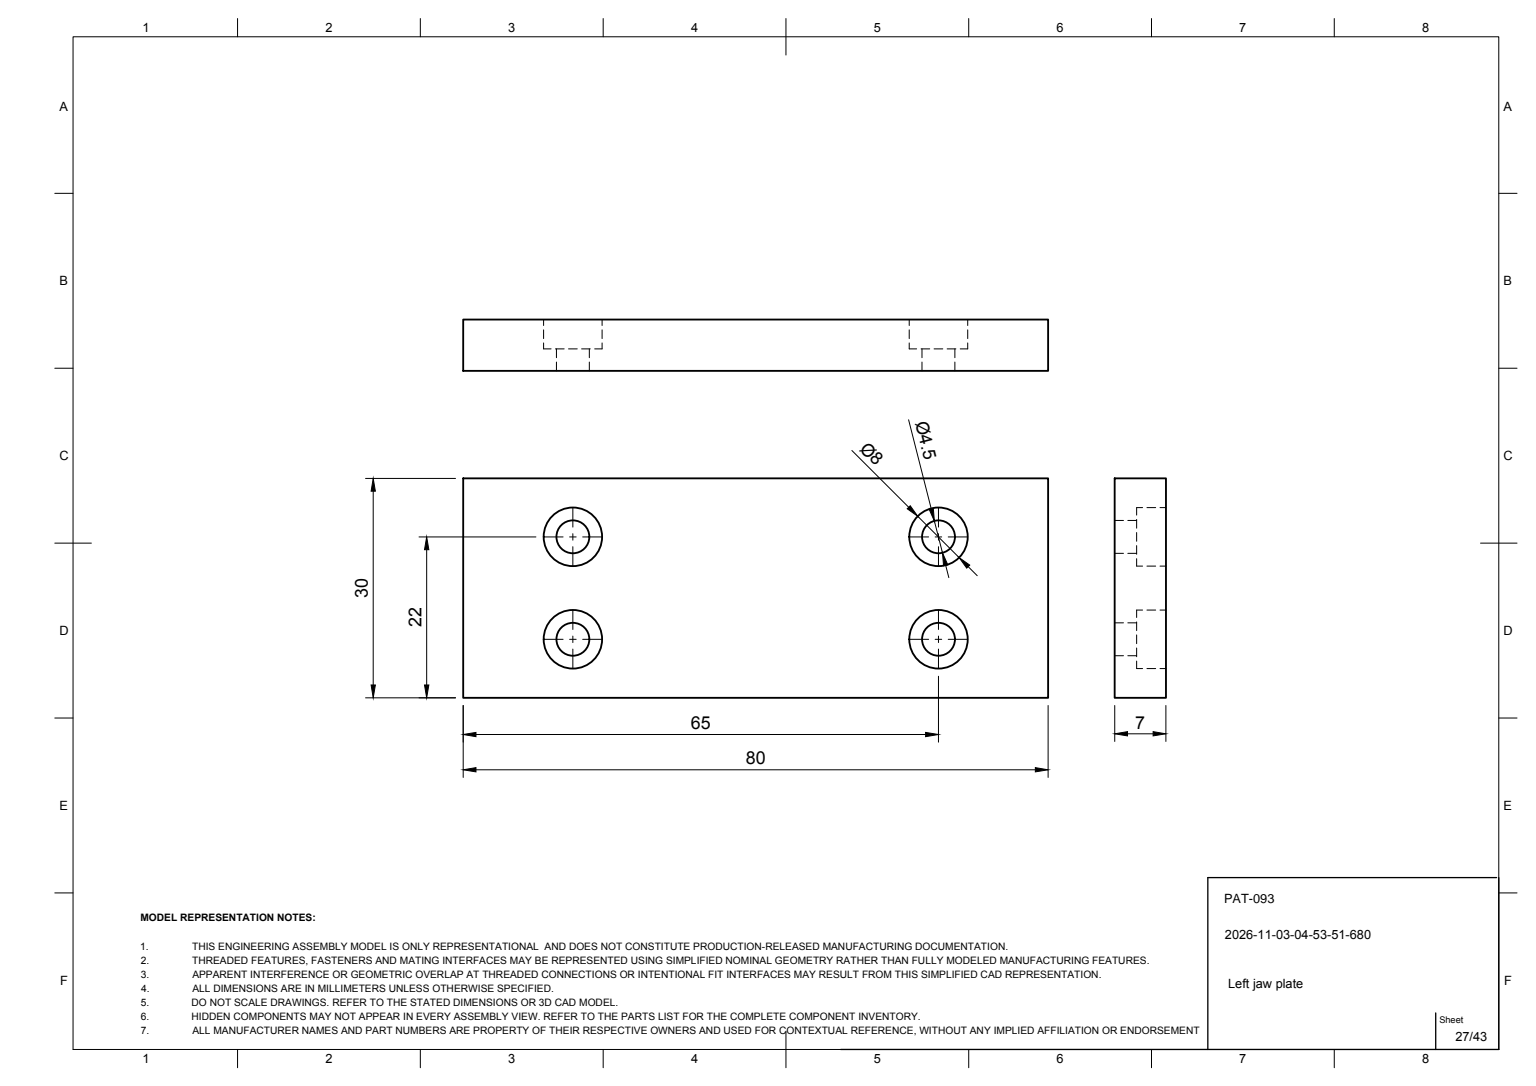
ISO-10303-21;
HEADER;
/* Generated by software containing ST-Developer
 * from STEP Tools, Inc. (www.steptools.com) 
 */

FILE_DESCRIPTION(
/* description */ ('Self-centering screw clamp'),
/* implementation_level */ '2;1');

FILE_NAME(
/* name */ 'Left jaw plate.step',
/* time_stamp */ '2026-10-28T03:25:31-07:00',
/* author */ (''),
/* organization */ (''),
/* preprocessor_version */ 'ST-DEVELOPER v20.2',
/* originating_system */ 'Autodesk Translation Framework v15.17.0.0',
/* authorisation */ '');

FILE_SCHEMA (('AUTOMOTIVE_DESIGN { 1 0 10303 214 3 1 1 }'));
ENDSEC;

DATA;
#10=MECHANICAL_DESIGN_GEOMETRIC_PRESENTATION_REPRESENTATION('',(#654),#16799);
#565=SHAPE_REPRESENTATION_RELATIONSHIP('SRR','None',#17040,#606);
#606=ADVANCED_BREP_SHAPE_REPRESENTATION('',(#702),#16778);
#654=STYLED_ITEM('',(#17340),#702);
#702=MANIFOLD_SOLID_BREP('Body1',#9105);
#904=FACE_BOUND('',#2255,.T.);
#905=FACE_BOUND('',#2258,.T.);
#906=FACE_BOUND('',#2261,.T.);
#907=FACE_BOUND('',#2264,.T.);
#908=FACE_BOUND('',#2271,.T.);
#909=FACE_BOUND('',#2272,.T.);
#910=FACE_BOUND('',#2273,.T.);
#911=FACE_BOUND('',#2274,.T.);
#912=FACE_BOUND('',#2277,.T.);
#913=FACE_BOUND('',#2278,.T.);
#914=FACE_BOUND('',#2279,.T.);
#915=FACE_BOUND('',#2280,.T.);
#1151=PLANE('',#10224);
#1152=PLANE('',#10229);
#1153=PLANE('',#10234);
#1154=PLANE('',#10239);
#1155=PLANE('',#10249);
#1156=PLANE('',#10250);
#1157=PLANE('',#10251);
#1158=PLANE('',#10252);
#1159=PLANE('',#10253);
#1160=PLANE('',#10254);
#1563=FACE_OUTER_BOUND('',#2253,.T.);
#1564=FACE_OUTER_BOUND('',#2254,.T.);
#1565=FACE_OUTER_BOUND('',#2256,.T.);
#1566=FACE_OUTER_BOUND('',#2257,.T.);
#1567=FACE_OUTER_BOUND('',#2259,.T.);
#1568=FACE_OUTER_BOUND('',#2260,.T.);
#1569=FACE_OUTER_BOUND('',#2262,.T.);
#1570=FACE_OUTER_BOUND('',#2263,.T.);
#1571=FACE_OUTER_BOUND('',#2265,.T.);
#1572=FACE_OUTER_BOUND('',#2266,.T.);
#1573=FACE_OUTER_BOUND('',#2267,.T.);
#1574=FACE_OUTER_BOUND('',#2268,.T.);
#1575=FACE_OUTER_BOUND('',#2269,.T.);
#1576=FACE_OUTER_BOUND('',#2270,.T.);
#1577=FACE_OUTER_BOUND('',#2275,.T.);
#1578=FACE_OUTER_BOUND('',#2276,.T.);
#1579=FACE_OUTER_BOUND('',#2281,.T.);
#1580=FACE_OUTER_BOUND('',#2282,.T.);
#2253=EDGE_LOOP('',(#7479,#7480,#7481,#7482));
#2254=EDGE_LOOP('',(#7483));
#2255=EDGE_LOOP('',(#7484));
#2256=EDGE_LOOP('',(#7485,#7486,#7487,#7488));
#2257=EDGE_LOOP('',(#7489));
#2258=EDGE_LOOP('',(#7490));
#2259=EDGE_LOOP('',(#7491,#7492,#7493,#7494));
#2260=EDGE_LOOP('',(#7495));
#2261=EDGE_LOOP('',(#7496));
#2262=EDGE_LOOP('',(#7497,#7498,#7499,#7500));
#2263=EDGE_LOOP('',(#7501));
#2264=EDGE_LOOP('',(#7502));
#2265=EDGE_LOOP('',(#7503,#7504,#7505,#7506));
#2266=EDGE_LOOP('',(#7507,#7508,#7509,#7510));
#2267=EDGE_LOOP('',(#7511,#7512,#7513,#7514));
#2268=EDGE_LOOP('',(#7515,#7516,#7517,#7518));
#2269=EDGE_LOOP('',(#7519,#7520,#7521,#7522));
#2270=EDGE_LOOP('',(#7523,#7524,#7525,#7526));
#2271=EDGE_LOOP('',(#7527));
#2272=EDGE_LOOP('',(#7528));
#2273=EDGE_LOOP('',(#7529));
#2274=EDGE_LOOP('',(#7530));
#2275=EDGE_LOOP('',(#7531,#7532,#7533,#7534));
#2276=EDGE_LOOP('',(#7535,#7536,#7537,#7538));
#2277=EDGE_LOOP('',(#7539));
#2278=EDGE_LOOP('',(#7540));
#2279=EDGE_LOOP('',(#7541));
#2280=EDGE_LOOP('',(#7542));
#2281=EDGE_LOOP('',(#7543,#7544,#7545,#7546));
#2282=EDGE_LOOP('',(#7547,#7548,#7549,#7550));
#2914=LINE('',#15518,#3487);
#2915=LINE('',#15527,#3488);
#2916=LINE('',#15536,#3489);
#2917=LINE('',#15545,#3490);
#2918=LINE('',#15553,#3491);
#2919=LINE('',#15557,#3492);
#2920=LINE('',#15561,#3493);
#2921=LINE('',#15565,#3494);
#2922=LINE('',#15569,#3495);
#2923=LINE('',#15571,#3496);
#2924=LINE('',#15573,#3497);
#2925=LINE('',#15574,#3498);
#2926=LINE('',#15577,#3499);
#2927=LINE('',#15579,#3500);
#2928=LINE('',#15580,#3501);
#2929=LINE('',#15583,#3502);
#2930=LINE('',#15585,#3503);
#2931=LINE('',#15586,#3504);
#2932=LINE('',#15588,#3505);
#2933=LINE('',#15589,#3506);
#3487=VECTOR('',#12381,0.4);
#3488=VECTOR('',#12392,0.4);
#3489=VECTOR('',#12403,0.4);
#3490=VECTOR('',#12414,0.4);
#3491=VECTOR('',#12425,0.225);
#3492=VECTOR('',#12430,0.225);
#3493=VECTOR('',#12435,0.225);
#3494=VECTOR('',#12440,0.225);
#3495=VECTOR('',#12443,1.);
#3496=VECTOR('',#12444,1.);
#3497=VECTOR('',#12445,1.);
#3498=VECTOR('',#12446,1.);
#3499=VECTOR('',#12449,1.);
#3500=VECTOR('',#12450,1.);
#3501=VECTOR('',#12451,1.);
#3502=VECTOR('',#12454,1.);
#3503=VECTOR('',#12455,1.);
#3504=VECTOR('',#12456,1.);
#3505=VECTOR('',#12459,1.);
#3506=VECTOR('',#12460,1.);
#4044=CIRCLE('',#10222,0.4);
#4045=CIRCLE('',#10223,0.4);
#4046=CIRCLE('',#10225,0.225);
#4047=CIRCLE('',#10227,0.4);
#4048=CIRCLE('',#10228,0.4);
#4049=CIRCLE('',#10230,0.225);
#4050=CIRCLE('',#10232,0.4);
#4051=CIRCLE('',#10233,0.4);
#4052=CIRCLE('',#10235,0.225);
#4053=CIRCLE('',#10237,0.4);
#4054=CIRCLE('',#10238,0.4);
#4055=CIRCLE('',#10240,0.225);
#4056=CIRCLE('',#10242,0.225);
#4057=CIRCLE('',#10244,0.225);
#4058=CIRCLE('',#10246,0.225);
#4059=CIRCLE('',#10248,0.225);
#4687=VERTEX_POINT('',#15515);
#4688=VERTEX_POINT('',#15517);
#4689=VERTEX_POINT('',#15521);
#4690=VERTEX_POINT('',#15524);
#4691=VERTEX_POINT('',#15526);
#4692=VERTEX_POINT('',#15530);
#4693=VERTEX_POINT('',#15533);
#4694=VERTEX_POINT('',#15535);
#4695=VERTEX_POINT('',#15539);
#4696=VERTEX_POINT('',#15542);
#4697=VERTEX_POINT('',#15544);
#4698=VERTEX_POINT('',#15548);
#4699=VERTEX_POINT('',#15551);
#4700=VERTEX_POINT('',#15555);
#4701=VERTEX_POINT('',#15559);
#4702=VERTEX_POINT('',#15563);
#4703=VERTEX_POINT('',#15567);
#4704=VERTEX_POINT('',#15568);
#4705=VERTEX_POINT('',#15570);
#4706=VERTEX_POINT('',#15572);
#4707=VERTEX_POINT('',#15576);
#4708=VERTEX_POINT('',#15578);
#4709=VERTEX_POINT('',#15582);
#4710=VERTEX_POINT('',#15584);
#5664=EDGE_CURVE('',#4687,#4687,#4044,.T.);
#5665=EDGE_CURVE('',#4687,#4688,#2914,.T.);
#5666=EDGE_CURVE('',#4688,#4688,#4045,.T.);
#5667=EDGE_CURVE('',#4689,#4689,#4046,.T.);
#5668=EDGE_CURVE('',#4690,#4690,#4047,.T.);
#5669=EDGE_CURVE('',#4690,#4691,#2915,.T.);
#5670=EDGE_CURVE('',#4691,#4691,#4048,.T.);
#5671=EDGE_CURVE('',#4692,#4692,#4049,.T.);
#5672=EDGE_CURVE('',#4693,#4693,#4050,.T.);
#5673=EDGE_CURVE('',#4693,#4694,#2916,.T.);
#5674=EDGE_CURVE('',#4694,#4694,#4051,.T.);
#5675=EDGE_CURVE('',#4695,#4695,#4052,.T.);
#5676=EDGE_CURVE('',#4696,#4696,#4053,.T.);
#5677=EDGE_CURVE('',#4696,#4697,#2917,.T.);
#5678=EDGE_CURVE('',#4697,#4697,#4054,.T.);
#5679=EDGE_CURVE('',#4698,#4698,#4055,.T.);
#5680=EDGE_CURVE('',#4699,#4699,#4056,.T.);
#5681=EDGE_CURVE('',#4699,#4689,#2918,.T.);
#5682=EDGE_CURVE('',#4700,#4700,#4057,.T.);
#5683=EDGE_CURVE('',#4700,#4692,#2919,.T.);
#5684=EDGE_CURVE('',#4701,#4701,#4058,.T.);
#5685=EDGE_CURVE('',#4701,#4695,#2920,.T.);
#5686=EDGE_CURVE('',#4702,#4702,#4059,.T.);
#5687=EDGE_CURVE('',#4702,#4698,#2921,.T.);
#5688=EDGE_CURVE('',#4703,#4704,#2922,.T.);
#5689=EDGE_CURVE('',#4704,#4705,#2923,.T.);
#5690=EDGE_CURVE('',#4706,#4705,#2924,.T.);
#5691=EDGE_CURVE('',#4703,#4706,#2925,.T.);
#5692=EDGE_CURVE('',#4707,#4703,#2926,.T.);
#5693=EDGE_CURVE('',#4708,#4706,#2927,.T.);
#5694=EDGE_CURVE('',#4707,#4708,#2928,.T.);
#5695=EDGE_CURVE('',#4709,#4707,#2929,.T.);
#5696=EDGE_CURVE('',#4710,#4708,#2930,.T.);
#5697=EDGE_CURVE('',#4709,#4710,#2931,.T.);
#5698=EDGE_CURVE('',#4704,#4709,#2932,.T.);
#5699=EDGE_CURVE('',#4705,#4710,#2933,.T.);
#7479=ORIENTED_EDGE('',*,*,#5664,.F.);
#7480=ORIENTED_EDGE('',*,*,#5665,.T.);
#7481=ORIENTED_EDGE('',*,*,#5666,.F.);
#7482=ORIENTED_EDGE('',*,*,#5665,.F.);
#7483=ORIENTED_EDGE('',*,*,#5664,.T.);
#7484=ORIENTED_EDGE('',*,*,#5667,.F.);
#7485=ORIENTED_EDGE('',*,*,#5668,.F.);
#7486=ORIENTED_EDGE('',*,*,#5669,.T.);
#7487=ORIENTED_EDGE('',*,*,#5670,.F.);
#7488=ORIENTED_EDGE('',*,*,#5669,.F.);
#7489=ORIENTED_EDGE('',*,*,#5668,.T.);
#7490=ORIENTED_EDGE('',*,*,#5671,.F.);
#7491=ORIENTED_EDGE('',*,*,#5672,.F.);
#7492=ORIENTED_EDGE('',*,*,#5673,.T.);
#7493=ORIENTED_EDGE('',*,*,#5674,.F.);
#7494=ORIENTED_EDGE('',*,*,#5673,.F.);
#7495=ORIENTED_EDGE('',*,*,#5672,.T.);
#7496=ORIENTED_EDGE('',*,*,#5675,.F.);
#7497=ORIENTED_EDGE('',*,*,#5676,.F.);
#7498=ORIENTED_EDGE('',*,*,#5677,.T.);
#7499=ORIENTED_EDGE('',*,*,#5678,.F.);
#7500=ORIENTED_EDGE('',*,*,#5677,.F.);
#7501=ORIENTED_EDGE('',*,*,#5676,.T.);
#7502=ORIENTED_EDGE('',*,*,#5679,.F.);
#7503=ORIENTED_EDGE('',*,*,#5680,.F.);
#7504=ORIENTED_EDGE('',*,*,#5681,.T.);
#7505=ORIENTED_EDGE('',*,*,#5667,.T.);
#7506=ORIENTED_EDGE('',*,*,#5681,.F.);
#7507=ORIENTED_EDGE('',*,*,#5682,.F.);
#7508=ORIENTED_EDGE('',*,*,#5683,.T.);
#7509=ORIENTED_EDGE('',*,*,#5671,.T.);
#7510=ORIENTED_EDGE('',*,*,#5683,.F.);
#7511=ORIENTED_EDGE('',*,*,#5684,.F.);
#7512=ORIENTED_EDGE('',*,*,#5685,.T.);
#7513=ORIENTED_EDGE('',*,*,#5675,.T.);
#7514=ORIENTED_EDGE('',*,*,#5685,.F.);
#7515=ORIENTED_EDGE('',*,*,#5686,.F.);
#7516=ORIENTED_EDGE('',*,*,#5687,.T.);
#7517=ORIENTED_EDGE('',*,*,#5679,.T.);
#7518=ORIENTED_EDGE('',*,*,#5687,.F.);
#7519=ORIENTED_EDGE('',*,*,#5688,.T.);
#7520=ORIENTED_EDGE('',*,*,#5689,.T.);
#7521=ORIENTED_EDGE('',*,*,#5690,.F.);
#7522=ORIENTED_EDGE('',*,*,#5691,.F.);
#7523=ORIENTED_EDGE('',*,*,#5692,.T.);
#7524=ORIENTED_EDGE('',*,*,#5691,.T.);
#7525=ORIENTED_EDGE('',*,*,#5693,.F.);
#7526=ORIENTED_EDGE('',*,*,#5694,.F.);
#7527=ORIENTED_EDGE('',*,*,#5678,.T.);
#7528=ORIENTED_EDGE('',*,*,#5674,.T.);
#7529=ORIENTED_EDGE('',*,*,#5670,.T.);
#7530=ORIENTED_EDGE('',*,*,#5666,.T.);
#7531=ORIENTED_EDGE('',*,*,#5695,.T.);
#7532=ORIENTED_EDGE('',*,*,#5694,.T.);
#7533=ORIENTED_EDGE('',*,*,#5696,.F.);
#7534=ORIENTED_EDGE('',*,*,#5697,.F.);
#7535=ORIENTED_EDGE('',*,*,#5698,.T.);
#7536=ORIENTED_EDGE('',*,*,#5697,.T.);
#7537=ORIENTED_EDGE('',*,*,#5699,.F.);
#7538=ORIENTED_EDGE('',*,*,#5689,.F.);
#7539=ORIENTED_EDGE('',*,*,#5680,.T.);
#7540=ORIENTED_EDGE('',*,*,#5682,.T.);
#7541=ORIENTED_EDGE('',*,*,#5684,.T.);
#7542=ORIENTED_EDGE('',*,*,#5686,.T.);
#7543=ORIENTED_EDGE('',*,*,#5699,.T.);
#7544=ORIENTED_EDGE('',*,*,#5696,.T.);
#7545=ORIENTED_EDGE('',*,*,#5693,.T.);
#7546=ORIENTED_EDGE('',*,*,#5690,.T.);
#7547=ORIENTED_EDGE('',*,*,#5698,.F.);
#7548=ORIENTED_EDGE('',*,*,#5688,.F.);
#7549=ORIENTED_EDGE('',*,*,#5692,.F.);
#7550=ORIENTED_EDGE('',*,*,#5695,.F.);
#8488=CYLINDRICAL_SURFACE('',#10221,0.4);
#8489=CYLINDRICAL_SURFACE('',#10226,0.4);
#8490=CYLINDRICAL_SURFACE('',#10231,0.4);
#8491=CYLINDRICAL_SURFACE('',#10236,0.4);
#8492=CYLINDRICAL_SURFACE('',#10241,0.225);
#8493=CYLINDRICAL_SURFACE('',#10243,0.225);
#8494=CYLINDRICAL_SURFACE('',#10245,0.225);
#8495=CYLINDRICAL_SURFACE('',#10247,0.225);
#8861=ADVANCED_FACE('',(#1563),#8488,.F.);
#8862=ADVANCED_FACE('',(#1564,#904),#1151,.T.);
#8863=ADVANCED_FACE('',(#1565),#8489,.F.);
#8864=ADVANCED_FACE('',(#1566,#905),#1152,.T.);
#8865=ADVANCED_FACE('',(#1567),#8490,.F.);
#8866=ADVANCED_FACE('',(#1568,#906),#1153,.T.);
#8867=ADVANCED_FACE('',(#1569),#8491,.F.);
#8868=ADVANCED_FACE('',(#1570,#907),#1154,.T.);
#8869=ADVANCED_FACE('',(#1571),#8492,.F.);
#8870=ADVANCED_FACE('',(#1572),#8493,.F.);
#8871=ADVANCED_FACE('',(#1573),#8494,.F.);
#8872=ADVANCED_FACE('',(#1574),#8495,.F.);
#8873=ADVANCED_FACE('',(#1575),#1155,.T.);
#8874=ADVANCED_FACE('',(#1576,#908,#909,#910,#911),#1156,.T.);
#8875=ADVANCED_FACE('',(#1577),#1157,.T.);
#8876=ADVANCED_FACE('',(#1578,#912,#913,#914,#915),#1158,.T.);
#8877=ADVANCED_FACE('',(#1579),#1159,.T.);
#8878=ADVANCED_FACE('',(#1580),#1160,.F.);
#9105=CLOSED_SHELL('',(#8861,#8862,#8863,#8864,#8865,#8866,#8867,#8868,
#8869,#8870,#8871,#8872,#8873,#8874,#8875,#8876,#8877,#8878));
#10220=AXIS2_PLACEMENT_3D('',#15513,#12375,#12376);
#10221=AXIS2_PLACEMENT_3D('',#15514,#12377,#12378);
#10222=AXIS2_PLACEMENT_3D('',#15516,#12379,#12380);
#10223=AXIS2_PLACEMENT_3D('',#15519,#12382,#12383);
#10224=AXIS2_PLACEMENT_3D('',#15520,#12384,#12385);
#10225=AXIS2_PLACEMENT_3D('',#15522,#12386,#12387);
#10226=AXIS2_PLACEMENT_3D('',#15523,#12388,#12389);
#10227=AXIS2_PLACEMENT_3D('',#15525,#12390,#12391);
#10228=AXIS2_PLACEMENT_3D('',#15528,#12393,#12394);
#10229=AXIS2_PLACEMENT_3D('',#15529,#12395,#12396);
#10230=AXIS2_PLACEMENT_3D('',#15531,#12397,#12398);
#10231=AXIS2_PLACEMENT_3D('',#15532,#12399,#12400);
#10232=AXIS2_PLACEMENT_3D('',#15534,#12401,#12402);
#10233=AXIS2_PLACEMENT_3D('',#15537,#12404,#12405);
#10234=AXIS2_PLACEMENT_3D('',#15538,#12406,#12407);
#10235=AXIS2_PLACEMENT_3D('',#15540,#12408,#12409);
#10236=AXIS2_PLACEMENT_3D('',#15541,#12410,#12411);
#10237=AXIS2_PLACEMENT_3D('',#15543,#12412,#12413);
#10238=AXIS2_PLACEMENT_3D('',#15546,#12415,#12416);
#10239=AXIS2_PLACEMENT_3D('',#15547,#12417,#12418);
#10240=AXIS2_PLACEMENT_3D('',#15549,#12419,#12420);
#10241=AXIS2_PLACEMENT_3D('',#15550,#12421,#12422);
#10242=AXIS2_PLACEMENT_3D('',#15552,#12423,#12424);
#10243=AXIS2_PLACEMENT_3D('',#15554,#12426,#12427);
#10244=AXIS2_PLACEMENT_3D('',#15556,#12428,#12429);
#10245=AXIS2_PLACEMENT_3D('',#15558,#12431,#12432);
#10246=AXIS2_PLACEMENT_3D('',#15560,#12433,#12434);
#10247=AXIS2_PLACEMENT_3D('',#15562,#12436,#12437);
#10248=AXIS2_PLACEMENT_3D('',#15564,#12438,#12439);
#10249=AXIS2_PLACEMENT_3D('',#15566,#12441,#12442);
#10250=AXIS2_PLACEMENT_3D('',#15575,#12447,#12448);
#10251=AXIS2_PLACEMENT_3D('',#15581,#12452,#12453);
#10252=AXIS2_PLACEMENT_3D('',#15587,#12457,#12458);
#10253=AXIS2_PLACEMENT_3D('',#15590,#12461,#12462);
#10254=AXIS2_PLACEMENT_3D('',#15591,#12463,#12464);
#12375=DIRECTION('axis',(0.,0.,1.));
#12376=DIRECTION('refdir',(1.,0.,0.));
#12377=DIRECTION('center_axis',(1.,0.,0.));
#12378=DIRECTION('ref_axis',(0.,0.,-1.));
#12379=DIRECTION('center_axis',(1.,0.,0.));
#12380=DIRECTION('ref_axis',(0.,0.,-1.));
#12381=DIRECTION('',(1.,0.,0.));
#12382=DIRECTION('center_axis',(-1.,0.,0.));
#12383=DIRECTION('ref_axis',(0.,0.,-1.));
#12384=DIRECTION('center_axis',(1.,0.,0.));
#12385=DIRECTION('ref_axis',(0.,0.,-1.));
#12386=DIRECTION('center_axis',(1.,0.,0.));
#12387=DIRECTION('ref_axis',(0.,0.,-1.));
#12388=DIRECTION('center_axis',(1.,0.,0.));
#12389=DIRECTION('ref_axis',(0.,0.,-1.));
#12390=DIRECTION('center_axis',(1.,0.,0.));
#12391=DIRECTION('ref_axis',(0.,0.,-1.));
#12392=DIRECTION('',(1.,0.,0.));
#12393=DIRECTION('center_axis',(-1.,0.,0.));
#12394=DIRECTION('ref_axis',(0.,0.,-1.));
#12395=DIRECTION('center_axis',(1.,0.,0.));
#12396=DIRECTION('ref_axis',(0.,0.,-1.));
#12397=DIRECTION('center_axis',(1.,0.,0.));
#12398=DIRECTION('ref_axis',(0.,0.,-1.));
#12399=DIRECTION('center_axis',(1.,0.,0.));
#12400=DIRECTION('ref_axis',(0.,0.,-1.));
#12401=DIRECTION('center_axis',(1.,0.,0.));
#12402=DIRECTION('ref_axis',(0.,0.,-1.));
#12403=DIRECTION('',(1.,0.,0.));
#12404=DIRECTION('center_axis',(-1.,0.,0.));
#12405=DIRECTION('ref_axis',(0.,0.,-1.));
#12406=DIRECTION('center_axis',(1.,0.,0.));
#12407=DIRECTION('ref_axis',(0.,0.,-1.));
#12408=DIRECTION('center_axis',(1.,0.,0.));
#12409=DIRECTION('ref_axis',(0.,0.,-1.));
#12410=DIRECTION('center_axis',(1.,0.,0.));
#12411=DIRECTION('ref_axis',(0.,0.,-1.));
#12412=DIRECTION('center_axis',(1.,0.,0.));
#12413=DIRECTION('ref_axis',(0.,0.,-1.));
#12414=DIRECTION('',(1.,0.,0.));
#12415=DIRECTION('center_axis',(-1.,0.,0.));
#12416=DIRECTION('ref_axis',(0.,0.,-1.));
#12417=DIRECTION('center_axis',(1.,0.,0.));
#12418=DIRECTION('ref_axis',(0.,0.,-1.));
#12419=DIRECTION('center_axis',(1.,0.,0.));
#12420=DIRECTION('ref_axis',(0.,0.,-1.));
#12421=DIRECTION('center_axis',(1.,0.,0.));
#12422=DIRECTION('ref_axis',(0.,0.,-1.));
#12423=DIRECTION('center_axis',(1.,0.,0.));
#12424=DIRECTION('ref_axis',(0.,0.,-1.));
#12425=DIRECTION('',(1.,0.,0.));
#12426=DIRECTION('center_axis',(1.,0.,0.));
#12427=DIRECTION('ref_axis',(0.,0.,-1.));
#12428=DIRECTION('center_axis',(1.,0.,0.));
#12429=DIRECTION('ref_axis',(0.,0.,-1.));
#12430=DIRECTION('',(1.,0.,0.));
#12431=DIRECTION('center_axis',(1.,0.,0.));
#12432=DIRECTION('ref_axis',(0.,0.,-1.));
#12433=DIRECTION('center_axis',(1.,0.,0.));
#12434=DIRECTION('ref_axis',(0.,0.,-1.));
#12435=DIRECTION('',(1.,0.,0.));
#12436=DIRECTION('center_axis',(1.,0.,0.));
#12437=DIRECTION('ref_axis',(0.,0.,-1.));
#12438=DIRECTION('center_axis',(1.,0.,0.));
#12439=DIRECTION('ref_axis',(0.,0.,-1.));
#12440=DIRECTION('',(1.,0.,0.));
#12441=DIRECTION('center_axis',(0.,1.,0.));
#12442=DIRECTION('ref_axis',(-1.,0.,0.));
#12443=DIRECTION('',(-1.,0.,0.));
#12444=DIRECTION('',(0.,0.,1.));
#12445=DIRECTION('',(-1.,0.,0.));
#12446=DIRECTION('',(0.,0.,1.));
#12447=DIRECTION('center_axis',(1.,0.,0.));
#12448=DIRECTION('ref_axis',(0.,1.,0.));
#12449=DIRECTION('',(0.,1.,0.));
#12450=DIRECTION('',(0.,1.,0.));
#12451=DIRECTION('',(0.,0.,1.));
#12452=DIRECTION('center_axis',(0.,-1.,0.));
#12453=DIRECTION('ref_axis',(1.,0.,0.));
#12454=DIRECTION('',(1.,0.,0.));
#12455=DIRECTION('',(1.,0.,0.));
#12456=DIRECTION('',(0.,0.,1.));
#12457=DIRECTION('center_axis',(-1.,0.,0.));
#12458=DIRECTION('ref_axis',(0.,-1.,0.));
#12459=DIRECTION('',(0.,-1.,0.));
#12460=DIRECTION('',(0.,-1.,0.));
#12461=DIRECTION('center_axis',(0.,0.,1.));
#12462=DIRECTION('ref_axis',(1.,0.,0.));
#12463=DIRECTION('center_axis',(0.,0.,1.));
#12464=DIRECTION('ref_axis',(1.,0.,0.));
#15513=CARTESIAN_POINT('',(0.,0.,0.));
#15514=CARTESIAN_POINT('Origin',(-5.2,2.5,7.8));
#15515=CARTESIAN_POINT('',(-5.2,2.5,8.2));
#15516=CARTESIAN_POINT('Origin',(-5.2,2.5,7.8));
#15517=CARTESIAN_POINT('',(-4.8,2.5,8.2));
#15518=CARTESIAN_POINT('',(-5.2,2.5,8.2));
#15519=CARTESIAN_POINT('Origin',(-4.8,2.5,7.8));
#15520=CARTESIAN_POINT('Origin',(-5.2,2.5,7.8));
#15521=CARTESIAN_POINT('',(-5.2,2.5,8.025));
#15522=CARTESIAN_POINT('Origin',(-5.2,2.5,7.8));
#15523=CARTESIAN_POINT('Origin',(-5.2,-2.5,9.2));
#15524=CARTESIAN_POINT('',(-5.2,-2.5,9.6));
#15525=CARTESIAN_POINT('Origin',(-5.2,-2.5,9.2));
#15526=CARTESIAN_POINT('',(-4.8,-2.5,9.6));
#15527=CARTESIAN_POINT('',(-5.2,-2.5,9.6));
#15528=CARTESIAN_POINT('Origin',(-4.8,-2.5,9.2));
#15529=CARTESIAN_POINT('Origin',(-5.2,-2.5,9.2));
#15530=CARTESIAN_POINT('',(-5.2,-2.5,9.425));
#15531=CARTESIAN_POINT('Origin',(-5.2,-2.5,9.2));
#15532=CARTESIAN_POINT('Origin',(-5.2,-2.5,7.8));
#15533=CARTESIAN_POINT('',(-5.2,-2.5,8.2));
#15534=CARTESIAN_POINT('Origin',(-5.2,-2.5,7.8));
#15535=CARTESIAN_POINT('',(-4.8,-2.5,8.2));
#15536=CARTESIAN_POINT('',(-5.2,-2.5,8.2));
#15537=CARTESIAN_POINT('Origin',(-4.8,-2.5,7.8));
#15538=CARTESIAN_POINT('Origin',(-5.2,-2.5,7.8));
#15539=CARTESIAN_POINT('',(-5.2,-2.5,8.025));
#15540=CARTESIAN_POINT('Origin',(-5.2,-2.5,7.8));
#15541=CARTESIAN_POINT('Origin',(-5.2,2.5,9.2));
#15542=CARTESIAN_POINT('',(-5.2,2.5,9.6));
#15543=CARTESIAN_POINT('Origin',(-5.2,2.5,9.2));
#15544=CARTESIAN_POINT('',(-4.8,2.5,9.6));
#15545=CARTESIAN_POINT('',(-5.2,2.5,9.6));
#15546=CARTESIAN_POINT('Origin',(-4.8,2.5,9.2));
#15547=CARTESIAN_POINT('Origin',(-5.2,2.5,9.2));
#15548=CARTESIAN_POINT('',(-5.2,2.5,9.425));
#15549=CARTESIAN_POINT('Origin',(-5.2,2.5,9.2));
#15550=CARTESIAN_POINT('Origin',(-5.6,2.5,7.8));
#15551=CARTESIAN_POINT('',(-5.5,2.5,8.025));
#15552=CARTESIAN_POINT('Origin',(-5.5,2.5,7.8));
#15553=CARTESIAN_POINT('',(-5.6,2.5,8.025));
#15554=CARTESIAN_POINT('Origin',(-5.6,-2.5,9.2));
#15555=CARTESIAN_POINT('',(-5.5,-2.5,9.425));
#15556=CARTESIAN_POINT('Origin',(-5.5,-2.5,9.2));
#15557=CARTESIAN_POINT('',(-5.6,-2.5,9.425));
#15558=CARTESIAN_POINT('Origin',(-5.6,-2.5,7.8));
#15559=CARTESIAN_POINT('',(-5.5,-2.5,8.025));
#15560=CARTESIAN_POINT('Origin',(-5.5,-2.5,7.8));
#15561=CARTESIAN_POINT('',(-5.6,-2.5,8.025));
#15562=CARTESIAN_POINT('Origin',(-5.6,2.5,9.2));
#15563=CARTESIAN_POINT('',(-5.5,2.5,9.425));
#15564=CARTESIAN_POINT('Origin',(-5.5,2.5,9.2));
#15565=CARTESIAN_POINT('',(-5.6,2.5,9.425));
#15566=CARTESIAN_POINT('Origin',(-4.8,4.,7.));
#15567=CARTESIAN_POINT('',(-4.8,4.,7.));
#15568=CARTESIAN_POINT('',(-5.5,4.,7.));
#15569=CARTESIAN_POINT('',(-4.8,4.,7.));
#15570=CARTESIAN_POINT('',(-5.5,4.,10.));
#15571=CARTESIAN_POINT('',(-5.5,4.,7.));
#15572=CARTESIAN_POINT('',(-4.8,4.,10.));
#15573=CARTESIAN_POINT('',(-4.8,4.,10.));
#15574=CARTESIAN_POINT('',(-4.8,4.,7.));
#15575=CARTESIAN_POINT('Origin',(-4.8,-4.,7.));
#15576=CARTESIAN_POINT('',(-4.8,-4.,7.));
#15577=CARTESIAN_POINT('',(-4.8,-4.,7.));
#15578=CARTESIAN_POINT('',(-4.8,-4.,10.));
#15579=CARTESIAN_POINT('',(-4.8,-4.,10.));
#15580=CARTESIAN_POINT('',(-4.8,-4.,7.));
#15581=CARTESIAN_POINT('Origin',(-5.5,-4.,7.));
#15582=CARTESIAN_POINT('',(-5.5,-4.,7.));
#15583=CARTESIAN_POINT('',(-5.5,-4.,7.));
#15584=CARTESIAN_POINT('',(-5.5,-4.,10.));
#15585=CARTESIAN_POINT('',(-5.5,-4.,10.));
#15586=CARTESIAN_POINT('',(-5.5,-4.,7.));
#15587=CARTESIAN_POINT('Origin',(-5.5,4.,7.));
#15588=CARTESIAN_POINT('',(-5.5,4.,7.));
#15589=CARTESIAN_POINT('',(-5.5,4.,10.));
#15590=CARTESIAN_POINT('Origin',(-5.15,0.,10.));
#15591=CARTESIAN_POINT('Origin',(-5.15,0.,7.));
#16729=UNCERTAINTY_MEASURE_WITH_UNIT(LENGTH_MEASURE(0.001),#16800,
'DISTANCE_ACCURACY_VALUE',
'Maximum model space distance between geometric entities at asserted c
onnectivities');
#16750=UNCERTAINTY_MEASURE_WITH_UNIT(LENGTH_MEASURE(0.001),#16800,
'DISTANCE_ACCURACY_VALUE',
'Maximum model space distance between geometric entities at asserted c
onnectivities');
#16778=(
GEOMETRIC_REPRESENTATION_CONTEXT(3)
GLOBAL_UNCERTAINTY_ASSIGNED_CONTEXT((#16729))
GLOBAL_UNIT_ASSIGNED_CONTEXT((#16800,#16802,#16803))
REPRESENTATION_CONTEXT('','3D')
);
#16799=(
GEOMETRIC_REPRESENTATION_CONTEXT(3)
GLOBAL_UNCERTAINTY_ASSIGNED_CONTEXT((#16750))
GLOBAL_UNIT_ASSIGNED_CONTEXT((#16800,#16802,#16803))
REPRESENTATION_CONTEXT('','3D')
);
#16800=(
LENGTH_UNIT()
NAMED_UNIT(*)
SI_UNIT(.CENTI.,.METRE.)
);
#16802=(
NAMED_UNIT(*)
PLANE_ANGLE_UNIT()
SI_UNIT($,.RADIAN.)
);
#16803=(
NAMED_UNIT(*)
SI_UNIT($,.STERADIAN.)
SOLID_ANGLE_UNIT()
);
#16831=SHAPE_DEFINITION_REPRESENTATION(#16884,#17040);
#16884=PRODUCT_DEFINITION_SHAPE('',$,#17089);
#17040=SHAPE_REPRESENTATION('',(#10220),#16778);
#17061=PRODUCT_DEFINITION_CONTEXT('part definition',#17207,'design');
#17089=PRODUCT_DEFINITION('Left jaw plate','Left jaw plate',#17137,#17061);
#17137=PRODUCT_DEFINITION_FORMATION('',$,#17236);
#17207=APPLICATION_CONTEXT(
'Core Data for Automotive Mechanical Design Process');
#17208=PRODUCT_CONTEXT('part definition',#17207,'mechanical');
#17236=PRODUCT('Left jaw plate','Left jaw plate','Left jaw plate',(#17208));
#17334=COLOUR_RGB('Off White',0.89,0.88,0.83);
#17335=FILL_AREA_STYLE_COLOUR('',#17334);
#17336=FILL_AREA_STYLE('',(#17335));
#17337=SURFACE_STYLE_FILL_AREA(#17336);
#17338=SURFACE_SIDE_STYLE('',(#17337));
#17339=SURFACE_STYLE_USAGE(.BOTH.,#17338);
#17340=PRESENTATION_STYLE_ASSIGNMENT((#17339));
ENDSEC;
END-ISO-10303-21;
